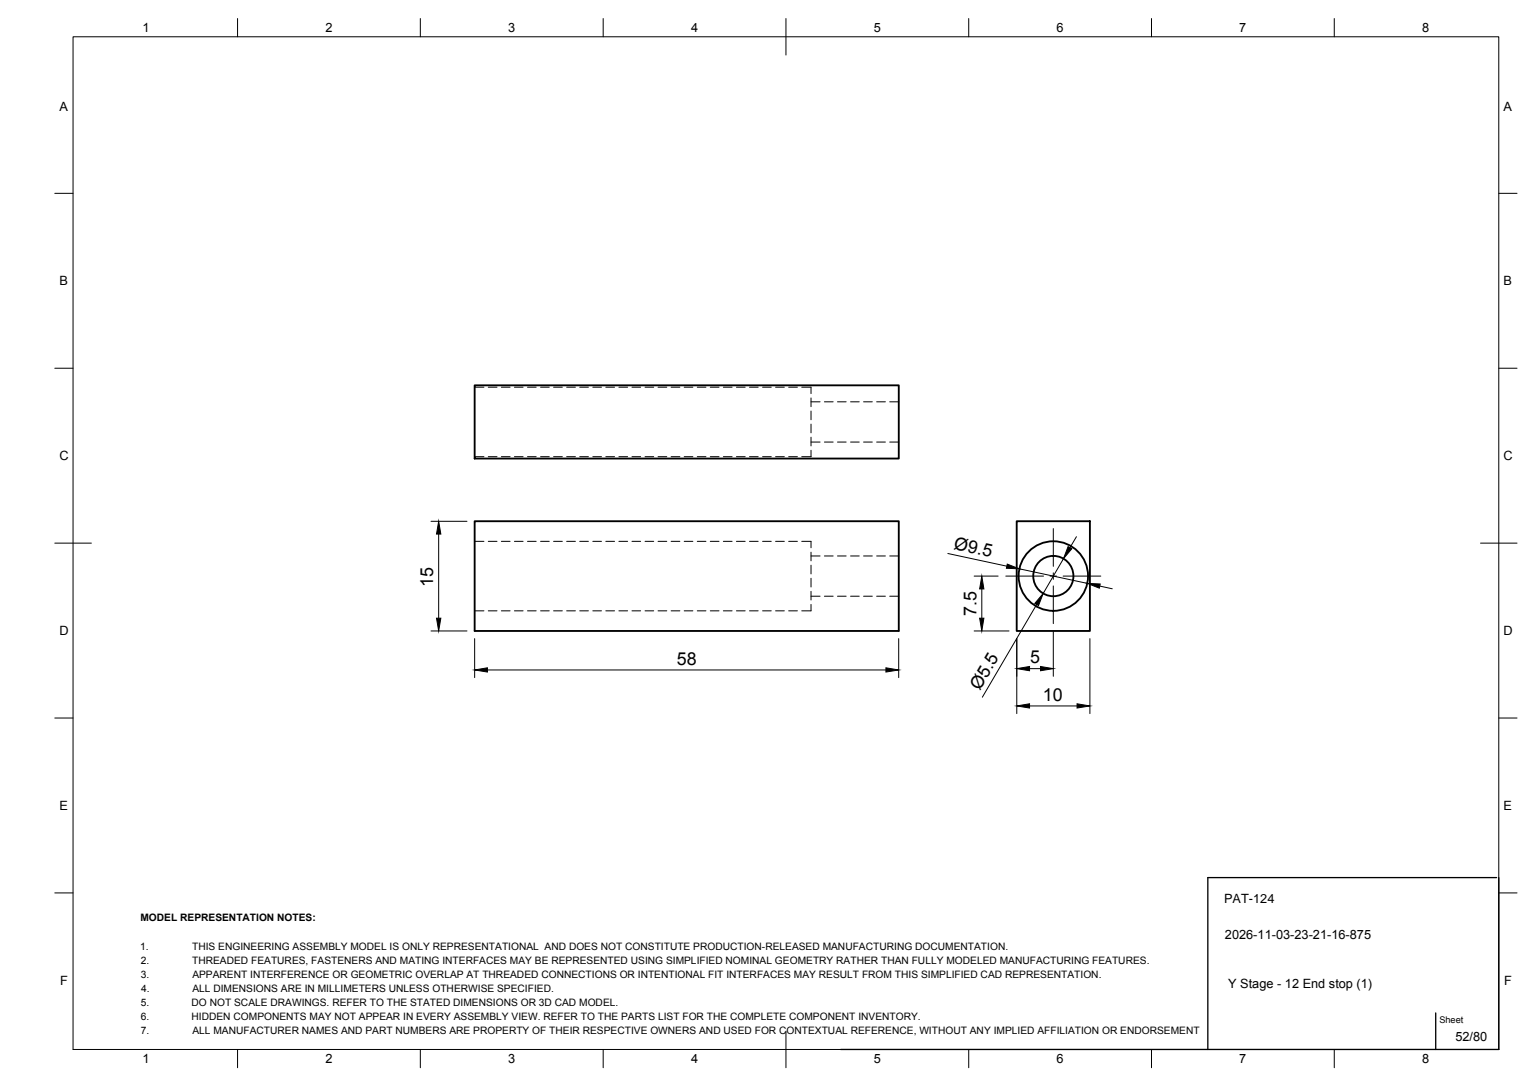
ISO-10303-21;
HEADER;
/* Generated by software containing ST-Developer
 * from STEP Tools, Inc. (www.steptools.com) 
 */

FILE_DESCRIPTION(
/* description */ ('XY cross-slide table'),
/* implementation_level */ '2;1');

FILE_NAME(
/* name */ 'Y Stage - 12 End stop (1).step',
/* time_stamp */ '2026-10-28T03:22:46-07:00',
/* author */ (''),
/* organization */ (''),
/* preprocessor_version */ 'ST-DEVELOPER v20.2',
/* originating_system */ 'Autodesk Translation Framework v15.17.0.0',
/* authorisation */ '');

FILE_SCHEMA (('AUTOMOTIVE_DESIGN { 1 0 10303 214 3 1 1 }'));
ENDSEC;

DATA;
#10=MECHANICAL_DESIGN_GEOMETRIC_PRESENTATION_REPRESENTATION('',(#1734),#62984);
#1553=SHAPE_REPRESENTATION_RELATIONSHIP('SRR','None',#63408,#1636);
#1636=ADVANCED_BREP_SHAPE_REPRESENTATION('',(#1843),#62945);
#1734=STYLED_ITEM('',(#63905),#1843);
#1843=MANIFOLD_SOLID_BREP('Body1',#23032);
#2186=FACE_BOUND('',#5255,.T.);
#2187=FACE_BOUND('',#5262,.T.);
#2188=FACE_BOUND('',#5264,.T.);
#2637=PLANE('',#25477);
#2638=PLANE('',#25481);
#2639=PLANE('',#25482);
#2640=PLANE('',#25483);
#2641=PLANE('',#25484);
#2642=PLANE('',#25485);
#2643=PLANE('',#25486);
#3640=FACE_OUTER_BOUND('',#5253,.T.);
#3641=FACE_OUTER_BOUND('',#5254,.T.);
#3642=FACE_OUTER_BOUND('',#5256,.T.);
#3643=FACE_OUTER_BOUND('',#5257,.T.);
#3644=FACE_OUTER_BOUND('',#5258,.T.);
#3645=FACE_OUTER_BOUND('',#5259,.T.);
#3646=FACE_OUTER_BOUND('',#5260,.T.);
#3647=FACE_OUTER_BOUND('',#5261,.T.);
#3648=FACE_OUTER_BOUND('',#5263,.T.);
#5253=EDGE_LOOP('',(#18472,#18473,#18474,#18475));
#5254=EDGE_LOOP('',(#18476));
#5255=EDGE_LOOP('',(#18477));
#5256=EDGE_LOOP('',(#18478,#18479,#18480,#18481));
#5257=EDGE_LOOP('',(#18482,#18483,#18484,#18485));
#5258=EDGE_LOOP('',(#18486,#18487,#18488,#18489));
#5259=EDGE_LOOP('',(#18490,#18491,#18492,#18493));
#5260=EDGE_LOOP('',(#18494,#18495,#18496,#18497));
#5261=EDGE_LOOP('',(#18498,#18499,#18500,#18501));
#5262=EDGE_LOOP('',(#18502));
#5263=EDGE_LOOP('',(#18503,#18504,#18505,#18506));
#5264=EDGE_LOOP('',(#18507));
#6779=LINE('',#48370,#8266);
#6780=LINE('',#48378,#8267);
#6781=LINE('',#48382,#8268);
#6782=LINE('',#48384,#8269);
#6783=LINE('',#48386,#8270);
#6784=LINE('',#48387,#8271);
#6785=LINE('',#48390,#8272);
#6786=LINE('',#48392,#8273);
#6787=LINE('',#48393,#8274);
#6788=LINE('',#48396,#8275);
#6789=LINE('',#48398,#8276);
#6790=LINE('',#48399,#8277);
#6791=LINE('',#48401,#8278);
#6792=LINE('',#48402,#8279);
#8266=VECTOR('',#30286,0.475000000000001);
#8267=VECTOR('',#30297,0.274999999999999);
#8268=VECTOR('',#30300,1.);
#8269=VECTOR('',#30301,1.);
#8270=VECTOR('',#30302,1.);
#8271=VECTOR('',#30303,1.);
#8272=VECTOR('',#30306,1.);
#8273=VECTOR('',#30307,1.);
#8274=VECTOR('',#30308,1.);
#8275=VECTOR('',#30311,1.);
#8276=VECTOR('',#30312,1.);
#8277=VECTOR('',#30313,1.);
#8278=VECTOR('',#30316,1.);
#8279=VECTOR('',#30317,1.);
#9447=CIRCLE('',#25475,0.475000000000001);
#9448=CIRCLE('',#25476,0.475000000000001);
#9449=CIRCLE('',#25478,0.274999999999999);
#9450=CIRCLE('',#25480,0.274999999999999);
#10969=VERTEX_POINT('',#48367);
#10970=VERTEX_POINT('',#48369);
#10971=VERTEX_POINT('',#48373);
#10972=VERTEX_POINT('',#48376);
#10973=VERTEX_POINT('',#48380);
#10974=VERTEX_POINT('',#48381);
#10975=VERTEX_POINT('',#48383);
#10976=VERTEX_POINT('',#48385);
#10977=VERTEX_POINT('',#48389);
#10978=VERTEX_POINT('',#48391);
#10979=VERTEX_POINT('',#48395);
#10980=VERTEX_POINT('',#48397);
#13620=EDGE_CURVE('',#10969,#10969,#9447,.T.);
#13621=EDGE_CURVE('',#10969,#10970,#6779,.T.);
#13622=EDGE_CURVE('',#10970,#10970,#9448,.T.);
#13623=EDGE_CURVE('',#10971,#10971,#9449,.T.);
#13624=EDGE_CURVE('',#10972,#10972,#9450,.T.);
#13625=EDGE_CURVE('',#10972,#10971,#6780,.T.);
#13626=EDGE_CURVE('',#10973,#10974,#6781,.T.);
#13627=EDGE_CURVE('',#10974,#10975,#6782,.T.);
#13628=EDGE_CURVE('',#10976,#10975,#6783,.T.);
#13629=EDGE_CURVE('',#10973,#10976,#6784,.T.);
#13630=EDGE_CURVE('',#10977,#10973,#6785,.T.);
#13631=EDGE_CURVE('',#10978,#10976,#6786,.T.);
#13632=EDGE_CURVE('',#10977,#10978,#6787,.T.);
#13633=EDGE_CURVE('',#10979,#10977,#6788,.T.);
#13634=EDGE_CURVE('',#10980,#10978,#6789,.T.);
#13635=EDGE_CURVE('',#10979,#10980,#6790,.T.);
#13636=EDGE_CURVE('',#10974,#10979,#6791,.T.);
#13637=EDGE_CURVE('',#10975,#10980,#6792,.T.);
#18472=ORIENTED_EDGE('',*,*,#13620,.F.);
#18473=ORIENTED_EDGE('',*,*,#13621,.T.);
#18474=ORIENTED_EDGE('',*,*,#13622,.F.);
#18475=ORIENTED_EDGE('',*,*,#13621,.F.);
#18476=ORIENTED_EDGE('',*,*,#13620,.T.);
#18477=ORIENTED_EDGE('',*,*,#13623,.F.);
#18478=ORIENTED_EDGE('',*,*,#13624,.F.);
#18479=ORIENTED_EDGE('',*,*,#13625,.T.);
#18480=ORIENTED_EDGE('',*,*,#13623,.T.);
#18481=ORIENTED_EDGE('',*,*,#13625,.F.);
#18482=ORIENTED_EDGE('',*,*,#13626,.T.);
#18483=ORIENTED_EDGE('',*,*,#13627,.T.);
#18484=ORIENTED_EDGE('',*,*,#13628,.F.);
#18485=ORIENTED_EDGE('',*,*,#13629,.F.);
#18486=ORIENTED_EDGE('',*,*,#13630,.T.);
#18487=ORIENTED_EDGE('',*,*,#13629,.T.);
#18488=ORIENTED_EDGE('',*,*,#13631,.F.);
#18489=ORIENTED_EDGE('',*,*,#13632,.F.);
#18490=ORIENTED_EDGE('',*,*,#13633,.T.);
#18491=ORIENTED_EDGE('',*,*,#13632,.T.);
#18492=ORIENTED_EDGE('',*,*,#13634,.F.);
#18493=ORIENTED_EDGE('',*,*,#13635,.F.);
#18494=ORIENTED_EDGE('',*,*,#13636,.T.);
#18495=ORIENTED_EDGE('',*,*,#13635,.T.);
#18496=ORIENTED_EDGE('',*,*,#13637,.F.);
#18497=ORIENTED_EDGE('',*,*,#13627,.F.);
#18498=ORIENTED_EDGE('',*,*,#13637,.T.);
#18499=ORIENTED_EDGE('',*,*,#13634,.T.);
#18500=ORIENTED_EDGE('',*,*,#13631,.T.);
#18501=ORIENTED_EDGE('',*,*,#13628,.T.);
#18502=ORIENTED_EDGE('',*,*,#13622,.T.);
#18503=ORIENTED_EDGE('',*,*,#13636,.F.);
#18504=ORIENTED_EDGE('',*,*,#13626,.F.);
#18505=ORIENTED_EDGE('',*,*,#13630,.F.);
#18506=ORIENTED_EDGE('',*,*,#13633,.F.);
#18507=ORIENTED_EDGE('',*,*,#13624,.T.);
#21406=CYLINDRICAL_SURFACE('',#25474,0.475000000000001);
#21407=CYLINDRICAL_SURFACE('',#25479,0.274999999999999);
#22421=ADVANCED_FACE('',(#3640),#21406,.F.);
#22422=ADVANCED_FACE('',(#3641,#2186),#2637,.T.);
#22423=ADVANCED_FACE('',(#3642),#21407,.F.);
#22424=ADVANCED_FACE('',(#3643),#2638,.T.);
#22425=ADVANCED_FACE('',(#3644),#2639,.T.);
#22426=ADVANCED_FACE('',(#3645),#2640,.T.);
#22427=ADVANCED_FACE('',(#3646),#2641,.T.);
#22428=ADVANCED_FACE('',(#3647,#2187),#2642,.T.);
#22429=ADVANCED_FACE('',(#3648,#2188),#2643,.F.);
#23032=CLOSED_SHELL('',(#22421,#22422,#22423,#22424,#22425,#22426,#22427,
#22428,#22429));
#25473=AXIS2_PLACEMENT_3D('',#48365,#30280,#30281);
#25474=AXIS2_PLACEMENT_3D('',#48366,#30282,#30283);
#25475=AXIS2_PLACEMENT_3D('',#48368,#30284,#30285);
#25476=AXIS2_PLACEMENT_3D('',#48371,#30287,#30288);
#25477=AXIS2_PLACEMENT_3D('',#48372,#30289,#30290);
#25478=AXIS2_PLACEMENT_3D('',#48374,#30291,#30292);
#25479=AXIS2_PLACEMENT_3D('',#48375,#30293,#30294);
#25480=AXIS2_PLACEMENT_3D('',#48377,#30295,#30296);
#25481=AXIS2_PLACEMENT_3D('',#48379,#30298,#30299);
#25482=AXIS2_PLACEMENT_3D('',#48388,#30304,#30305);
#25483=AXIS2_PLACEMENT_3D('',#48394,#30309,#30310);
#25484=AXIS2_PLACEMENT_3D('',#48400,#30314,#30315);
#25485=AXIS2_PLACEMENT_3D('',#48403,#30318,#30319);
#25486=AXIS2_PLACEMENT_3D('',#48404,#30320,#30321);
#30280=DIRECTION('axis',(0.,0.,1.));
#30281=DIRECTION('refdir',(1.,0.,0.));
#30282=DIRECTION('center_axis',(0.,0.,1.));
#30283=DIRECTION('ref_axis',(1.,0.,0.));
#30284=DIRECTION('center_axis',(0.,0.,1.));
#30285=DIRECTION('ref_axis',(1.,0.,0.));
#30286=DIRECTION('',(0.,0.,1.));
#30287=DIRECTION('center_axis',(0.,0.,-1.));
#30288=DIRECTION('ref_axis',(1.,0.,0.));
#30289=DIRECTION('center_axis',(0.,0.,1.));
#30290=DIRECTION('ref_axis',(1.,0.,0.));
#30291=DIRECTION('center_axis',(0.,0.,1.));
#30292=DIRECTION('ref_axis',(1.,0.,0.));
#30293=DIRECTION('center_axis',(0.,0.,1.));
#30294=DIRECTION('ref_axis',(1.,0.,0.));
#30295=DIRECTION('center_axis',(0.,0.,1.));
#30296=DIRECTION('ref_axis',(1.,0.,0.));
#30297=DIRECTION('',(0.,0.,1.));
#30298=DIRECTION('center_axis',(0.,1.,0.));
#30299=DIRECTION('ref_axis',(-1.,0.,0.));
#30300=DIRECTION('',(-1.,0.,0.));
#30301=DIRECTION('',(0.,0.,1.));
#30302=DIRECTION('',(-1.,0.,0.));
#30303=DIRECTION('',(0.,0.,1.));
#30304=DIRECTION('center_axis',(1.,0.,0.));
#30305=DIRECTION('ref_axis',(0.,1.,0.));
#30306=DIRECTION('',(0.,1.,0.));
#30307=DIRECTION('',(0.,1.,0.));
#30308=DIRECTION('',(0.,0.,1.));
#30309=DIRECTION('center_axis',(0.,-1.,0.));
#30310=DIRECTION('ref_axis',(1.,0.,0.));
#30311=DIRECTION('',(1.,0.,0.));
#30312=DIRECTION('',(1.,0.,0.));
#30313=DIRECTION('',(0.,0.,1.));
#30314=DIRECTION('center_axis',(-1.,0.,0.));
#30315=DIRECTION('ref_axis',(0.,-1.,0.));
#30316=DIRECTION('',(0.,-1.,0.));
#30317=DIRECTION('',(0.,-1.,0.));
#30318=DIRECTION('center_axis',(0.,0.,1.));
#30319=DIRECTION('ref_axis',(1.,0.,0.));
#30320=DIRECTION('center_axis',(0.,0.,1.));
#30321=DIRECTION('ref_axis',(1.,0.,0.));
#48365=CARTESIAN_POINT('',(0.,0.,0.));
#48366=CARTESIAN_POINT('Origin',(23.5,-9.25,2.4));
#48367=CARTESIAN_POINT('',(23.025,-9.25,2.4));
#48368=CARTESIAN_POINT('Origin',(23.5,-9.25,2.4));
#48369=CARTESIAN_POINT('',(23.025,-9.25,7.));
#48370=CARTESIAN_POINT('',(23.025,-9.25,2.4));
#48371=CARTESIAN_POINT('Origin',(23.5,-9.25,7.));
#48372=CARTESIAN_POINT('Origin',(23.5,-9.25,2.4));
#48373=CARTESIAN_POINT('',(23.225,-9.25,2.4));
#48374=CARTESIAN_POINT('Origin',(23.5,-9.25,2.4));
#48375=CARTESIAN_POINT('Origin',(23.5,-9.25,1.1));
#48376=CARTESIAN_POINT('',(23.225,-9.25,1.2));
#48377=CARTESIAN_POINT('Origin',(23.5,-9.25,1.2));
#48378=CARTESIAN_POINT('',(23.225,-9.25,1.1));
#48379=CARTESIAN_POINT('Origin',(24.,-8.5,1.2));
#48380=CARTESIAN_POINT('',(24.,-8.5,1.2));
#48381=CARTESIAN_POINT('',(23.,-8.5,1.2));
#48382=CARTESIAN_POINT('',(24.,-8.5,1.2));
#48383=CARTESIAN_POINT('',(23.,-8.5,7.));
#48384=CARTESIAN_POINT('',(23.,-8.5,1.2));
#48385=CARTESIAN_POINT('',(24.,-8.5,7.));
#48386=CARTESIAN_POINT('',(24.,-8.5,7.));
#48387=CARTESIAN_POINT('',(24.,-8.5,1.2));
#48388=CARTESIAN_POINT('Origin',(24.,-10.,1.2));
#48389=CARTESIAN_POINT('',(24.,-10.,1.2));
#48390=CARTESIAN_POINT('',(24.,-10.,1.2));
#48391=CARTESIAN_POINT('',(24.,-10.,7.));
#48392=CARTESIAN_POINT('',(24.,-10.,7.));
#48393=CARTESIAN_POINT('',(24.,-10.,1.2));
#48394=CARTESIAN_POINT('Origin',(23.,-10.,1.2));
#48395=CARTESIAN_POINT('',(23.,-10.,1.2));
#48396=CARTESIAN_POINT('',(23.,-10.,1.2));
#48397=CARTESIAN_POINT('',(23.,-10.,7.));
#48398=CARTESIAN_POINT('',(23.,-10.,7.));
#48399=CARTESIAN_POINT('',(23.,-10.,1.2));
#48400=CARTESIAN_POINT('Origin',(23.,-8.5,1.2));
#48401=CARTESIAN_POINT('',(23.,-8.5,1.2));
#48402=CARTESIAN_POINT('',(23.,-8.5,7.));
#48403=CARTESIAN_POINT('Origin',(23.5,-9.25,7.));
#48404=CARTESIAN_POINT('Origin',(23.5,-9.25,1.2));
#62846=UNCERTAINTY_MEASURE_WITH_UNIT(LENGTH_MEASURE(0.001),#62985,
'DISTANCE_ACCURACY_VALUE',
'Maximum model space distance between geometric entities at asserted c
onnectivities');
#62885=UNCERTAINTY_MEASURE_WITH_UNIT(LENGTH_MEASURE(0.001),#62985,
'DISTANCE_ACCURACY_VALUE',
'Maximum model space distance between geometric entities at asserted c
onnectivities');
#62945=(
GEOMETRIC_REPRESENTATION_CONTEXT(3)
GLOBAL_UNCERTAINTY_ASSIGNED_CONTEXT((#62846))
GLOBAL_UNIT_ASSIGNED_CONTEXT((#62985,#62987,#62988))
REPRESENTATION_CONTEXT('','3D')
);
#62984=(
GEOMETRIC_REPRESENTATION_CONTEXT(3)
GLOBAL_UNCERTAINTY_ASSIGNED_CONTEXT((#62885))
GLOBAL_UNIT_ASSIGNED_CONTEXT((#62985,#62987,#62988))
REPRESENTATION_CONTEXT('','3D')
);
#62985=(
LENGTH_UNIT()
NAMED_UNIT(*)
SI_UNIT(.CENTI.,.METRE.)
);
#62987=(
NAMED_UNIT(*)
PLANE_ANGLE_UNIT()
SI_UNIT($,.RADIAN.)
);
#62988=(
NAMED_UNIT(*)
SI_UNIT($,.STERADIAN.)
SOLID_ANGLE_UNIT()
);
#63048=SHAPE_DEFINITION_REPRESENTATION(#63226,#63408);
#63226=PRODUCT_DEFINITION_SHAPE('',$,#63507);
#63408=SHAPE_REPRESENTATION('',(#25473),#62945);
#63447=PRODUCT_DEFINITION_CONTEXT('part definition',#63743,'design');
#63507=PRODUCT_DEFINITION('Y Stage - 12 End stop (1)',
'Y Stage - 12 End stop (1)',#63605,#63447);
#63605=PRODUCT_DEFINITION_FORMATION('',$,#63804);
#63743=APPLICATION_CONTEXT(
'Core Data for Automotive Mechanical Design Process');
#63744=PRODUCT_CONTEXT('part definition',#63743,'mechanical');
#63804=PRODUCT('Y Stage - 12 End stop (1)','Y Stage - 12 End stop (1)',
'Y Stage - 12 End stop (1)',(#63744));
#63899=COLOUR_RGB('Sky Blue',0.24,0.69,0.87);
#63900=FILL_AREA_STYLE_COLOUR('',#63899);
#63901=FILL_AREA_STYLE('',(#63900));
#63902=SURFACE_STYLE_FILL_AREA(#63901);
#63903=SURFACE_SIDE_STYLE('',(#63902));
#63904=SURFACE_STYLE_USAGE(.BOTH.,#63903);
#63905=PRESENTATION_STYLE_ASSIGNMENT((#63904));
ENDSEC;
END-ISO-10303-21;
